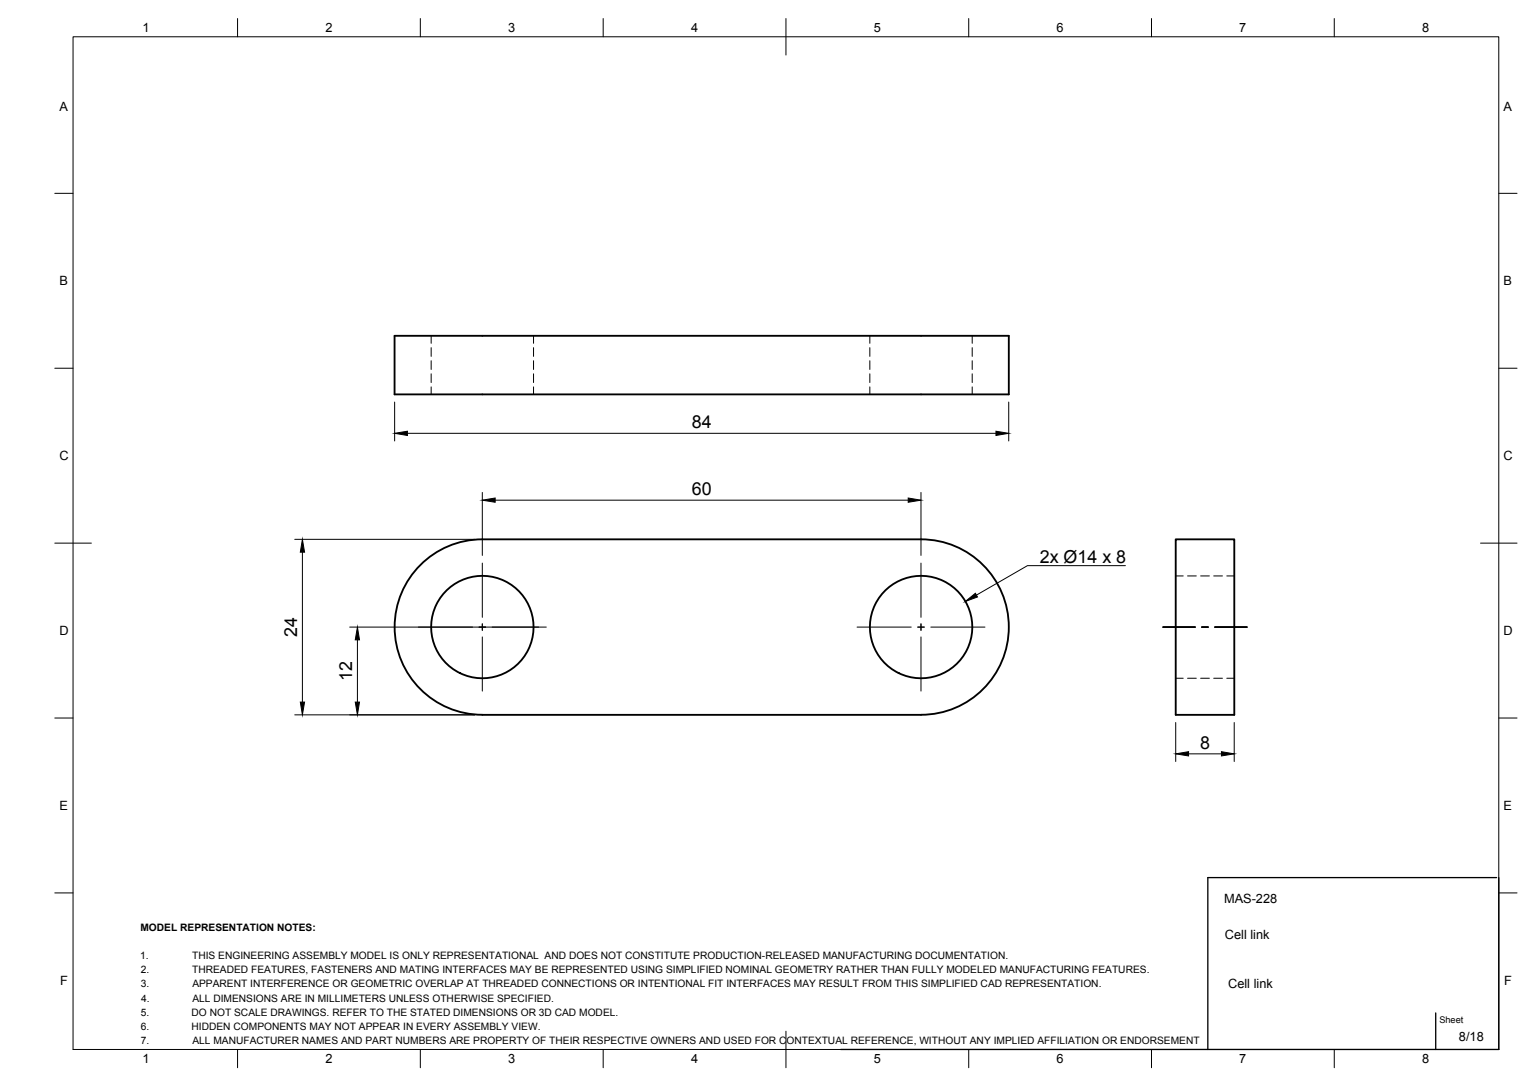
ISO-10303-21;
HEADER;
/* Generated by software containing ST-Developer
 * from STEP Tools, Inc. (www.steptools.com) 
 */

FILE_DESCRIPTION(
/* description */ ('Independent Peaucellier-Lipkin straight-line linkage. Radius arms 100
 mm, inversion-cell links 60 mm, crank radius and fixed-pivot spacing 
32 mm. Inversion constant 6400 mm squared, nominal output straight lin
e X=100 mm. Overhead bearing bridge clears the layered moving links. N
o accuracy or load rating assigned.'),
/* implementation_level */ '2;1');

FILE_NAME(
/* name */ 'Cell link.step',
/* time_stamp */ '2026-11-09T18:06:16-08:00',
/* author */ (''),
/* organization */ (''),
/* preprocessor_version */ 'ST-DEVELOPER v20.2',
/* originating_system */ 'Autodesk Translation Framework v15.17.0.0',
/* authorisation */ '');

FILE_SCHEMA (('AUTOMOTIVE_DESIGN { 1 0 10303 214 3 1 1 }'));
ENDSEC;

DATA;
#10=MECHANICAL_DESIGN_GEOMETRIC_PRESENTATION_REPRESENTATION('',(#288),#3581);
#254=SHAPE_REPRESENTATION_RELATIONSHIP('SRR','None',#3688,#271);
#271=ADVANCED_BREP_SHAPE_REPRESENTATION('',(#305),#3570);
#288=STYLED_ITEM('',(#3781),#305);
#305=MANIFOLD_SOLID_BREP('Body1',#1874);
#338=FACE_BOUND('',#606,.T.);
#339=FACE_BOUND('',#607,.T.);
#340=FACE_BOUND('',#609,.T.);
#341=FACE_BOUND('',#610,.T.);
#388=PLANE('',#2162);
#389=PLANE('',#2166);
#390=PLANE('',#2170);
#391=PLANE('',#2171);
#466=FACE_OUTER_BOUND('',#599,.T.);
#467=FACE_OUTER_BOUND('',#600,.T.);
#468=FACE_OUTER_BOUND('',#601,.T.);
#469=FACE_OUTER_BOUND('',#602,.T.);
#470=FACE_OUTER_BOUND('',#603,.T.);
#471=FACE_OUTER_BOUND('',#604,.T.);
#472=FACE_OUTER_BOUND('',#605,.T.);
#473=FACE_OUTER_BOUND('',#608,.T.);
#599=EDGE_LOOP('',(#1490,#1491,#1492,#1493));
#600=EDGE_LOOP('',(#1494,#1495,#1496,#1497));
#601=EDGE_LOOP('',(#1498,#1499,#1500,#1501));
#602=EDGE_LOOP('',(#1502,#1503,#1504,#1505));
#603=EDGE_LOOP('',(#1506,#1507,#1508,#1509));
#604=EDGE_LOOP('',(#1510,#1511,#1512,#1513));
#605=EDGE_LOOP('',(#1514,#1515,#1516,#1517));
#606=EDGE_LOOP('',(#1518));
#607=EDGE_LOOP('',(#1519));
#608=EDGE_LOOP('',(#1520,#1521,#1522,#1523));
#609=EDGE_LOOP('',(#1524));
#610=EDGE_LOOP('',(#1525));
#748=LINE('',#3227,#846);
#749=LINE('',#3233,#847);
#750=LINE('',#3238,#848);
#751=LINE('',#3240,#849);
#752=LINE('',#3242,#850);
#753=LINE('',#3243,#851);
#754=LINE('',#3249,#852);
#755=LINE('',#3252,#853);
#756=LINE('',#3254,#854);
#757=LINE('',#3255,#855);
#846=VECTOR('',#2582,7.);
#847=VECTOR('',#2589,7.);
#848=VECTOR('',#2594,10.);
#849=VECTOR('',#2595,10.);
#850=VECTOR('',#2596,10.);
#851=VECTOR('',#2597,10.);
#852=VECTOR('',#2604,10.);
#853=VECTOR('',#2607,10.);
#854=VECTOR('',#2608,10.);
#855=VECTOR('',#2609,10.);
#925=CIRCLE('',#2157,7.);
#926=CIRCLE('',#2158,7.);
#927=CIRCLE('',#2160,7.);
#928=CIRCLE('',#2161,7.);
#929=CIRCLE('',#2164,12.);
#930=CIRCLE('',#2165,12.);
#931=CIRCLE('',#2168,12.);
#932=CIRCLE('',#2169,12.);
#1047=VERTEX_POINT('',#3224);
#1048=VERTEX_POINT('',#3226);
#1049=VERTEX_POINT('',#3230);
#1050=VERTEX_POINT('',#3232);
#1051=VERTEX_POINT('',#3236);
#1052=VERTEX_POINT('',#3237);
#1053=VERTEX_POINT('',#3239);
#1054=VERTEX_POINT('',#3241);
#1055=VERTEX_POINT('',#3245);
#1056=VERTEX_POINT('',#3247);
#1057=VERTEX_POINT('',#3251);
#1058=VERTEX_POINT('',#3253);
#1207=EDGE_CURVE('',#1047,#1047,#925,.T.);
#1208=EDGE_CURVE('',#1047,#1048,#748,.T.);
#1209=EDGE_CURVE('',#1048,#1048,#926,.T.);
#1210=EDGE_CURVE('',#1049,#1049,#927,.T.);
#1211=EDGE_CURVE('',#1049,#1050,#749,.T.);
#1212=EDGE_CURVE('',#1050,#1050,#928,.T.);
#1213=EDGE_CURVE('',#1051,#1052,#750,.T.);
#1214=EDGE_CURVE('',#1052,#1053,#751,.T.);
#1215=EDGE_CURVE('',#1054,#1053,#752,.T.);
#1216=EDGE_CURVE('',#1051,#1054,#753,.T.);
#1217=EDGE_CURVE('',#1055,#1051,#929,.T.);
#1218=EDGE_CURVE('',#1056,#1054,#930,.T.);
#1219=EDGE_CURVE('',#1055,#1056,#754,.T.);
#1220=EDGE_CURVE('',#1057,#1055,#755,.T.);
#1221=EDGE_CURVE('',#1058,#1056,#756,.T.);
#1222=EDGE_CURVE('',#1057,#1058,#757,.T.);
#1223=EDGE_CURVE('',#1052,#1057,#931,.T.);
#1224=EDGE_CURVE('',#1053,#1058,#932,.T.);
#1490=ORIENTED_EDGE('',*,*,#1207,.F.);
#1491=ORIENTED_EDGE('',*,*,#1208,.T.);
#1492=ORIENTED_EDGE('',*,*,#1209,.F.);
#1493=ORIENTED_EDGE('',*,*,#1208,.F.);
#1494=ORIENTED_EDGE('',*,*,#1210,.F.);
#1495=ORIENTED_EDGE('',*,*,#1211,.T.);
#1496=ORIENTED_EDGE('',*,*,#1212,.F.);
#1497=ORIENTED_EDGE('',*,*,#1211,.F.);
#1498=ORIENTED_EDGE('',*,*,#1213,.T.);
#1499=ORIENTED_EDGE('',*,*,#1214,.T.);
#1500=ORIENTED_EDGE('',*,*,#1215,.F.);
#1501=ORIENTED_EDGE('',*,*,#1216,.F.);
#1502=ORIENTED_EDGE('',*,*,#1217,.T.);
#1503=ORIENTED_EDGE('',*,*,#1216,.T.);
#1504=ORIENTED_EDGE('',*,*,#1218,.F.);
#1505=ORIENTED_EDGE('',*,*,#1219,.F.);
#1506=ORIENTED_EDGE('',*,*,#1220,.T.);
#1507=ORIENTED_EDGE('',*,*,#1219,.T.);
#1508=ORIENTED_EDGE('',*,*,#1221,.F.);
#1509=ORIENTED_EDGE('',*,*,#1222,.F.);
#1510=ORIENTED_EDGE('',*,*,#1223,.T.);
#1511=ORIENTED_EDGE('',*,*,#1222,.T.);
#1512=ORIENTED_EDGE('',*,*,#1224,.F.);
#1513=ORIENTED_EDGE('',*,*,#1214,.F.);
#1514=ORIENTED_EDGE('',*,*,#1224,.T.);
#1515=ORIENTED_EDGE('',*,*,#1221,.T.);
#1516=ORIENTED_EDGE('',*,*,#1218,.T.);
#1517=ORIENTED_EDGE('',*,*,#1215,.T.);
#1518=ORIENTED_EDGE('',*,*,#1207,.T.);
#1519=ORIENTED_EDGE('',*,*,#1210,.T.);
#1520=ORIENTED_EDGE('',*,*,#1223,.F.);
#1521=ORIENTED_EDGE('',*,*,#1213,.F.);
#1522=ORIENTED_EDGE('',*,*,#1217,.F.);
#1523=ORIENTED_EDGE('',*,*,#1220,.F.);
#1524=ORIENTED_EDGE('',*,*,#1209,.T.);
#1525=ORIENTED_EDGE('',*,*,#1212,.T.);
#1725=CYLINDRICAL_SURFACE('',#2156,7.);
#1726=CYLINDRICAL_SURFACE('',#2159,7.);
#1727=CYLINDRICAL_SURFACE('',#2163,12.);
#1728=CYLINDRICAL_SURFACE('',#2167,12.);
#1798=ADVANCED_FACE('',(#466),#1725,.F.);
#1799=ADVANCED_FACE('',(#467),#1726,.F.);
#1800=ADVANCED_FACE('',(#468),#388,.T.);
#1801=ADVANCED_FACE('',(#469),#1727,.T.);
#1802=ADVANCED_FACE('',(#470),#389,.T.);
#1803=ADVANCED_FACE('',(#471),#1728,.T.);
#1804=ADVANCED_FACE('',(#472,#338,#339),#390,.T.);
#1805=ADVANCED_FACE('',(#473,#340,#341),#391,.F.);
#1874=CLOSED_SHELL('',(#1798,#1799,#1800,#1801,#1802,#1803,#1804,#1805));
#2155=AXIS2_PLACEMENT_3D('',#3222,#2576,#2577);
#2156=AXIS2_PLACEMENT_3D('',#3223,#2578,#2579);
#2157=AXIS2_PLACEMENT_3D('',#3225,#2580,#2581);
#2158=AXIS2_PLACEMENT_3D('',#3228,#2583,#2584);
#2159=AXIS2_PLACEMENT_3D('',#3229,#2585,#2586);
#2160=AXIS2_PLACEMENT_3D('',#3231,#2587,#2588);
#2161=AXIS2_PLACEMENT_3D('',#3234,#2590,#2591);
#2162=AXIS2_PLACEMENT_3D('',#3235,#2592,#2593);
#2163=AXIS2_PLACEMENT_3D('',#3244,#2598,#2599);
#2164=AXIS2_PLACEMENT_3D('',#3246,#2600,#2601);
#2165=AXIS2_PLACEMENT_3D('',#3248,#2602,#2603);
#2166=AXIS2_PLACEMENT_3D('',#3250,#2605,#2606);
#2167=AXIS2_PLACEMENT_3D('',#3256,#2610,#2611);
#2168=AXIS2_PLACEMENT_3D('',#3257,#2612,#2613);
#2169=AXIS2_PLACEMENT_3D('',#3258,#2614,#2615);
#2170=AXIS2_PLACEMENT_3D('',#3259,#2616,#2617);
#2171=AXIS2_PLACEMENT_3D('',#3260,#2618,#2619);
#2576=DIRECTION('axis',(0.,0.,1.));
#2577=DIRECTION('refdir',(1.,0.,0.));
#2578=DIRECTION('center_axis',(0.,0.,-1.));
#2579=DIRECTION('ref_axis',(1.,0.,0.));
#2580=DIRECTION('center_axis',(0.,0.,-1.));
#2581=DIRECTION('ref_axis',(1.,0.,0.));
#2582=DIRECTION('',(0.,0.,-1.));
#2583=DIRECTION('center_axis',(0.,0.,1.));
#2584=DIRECTION('ref_axis',(1.,0.,0.));
#2585=DIRECTION('center_axis',(0.,0.,-1.));
#2586=DIRECTION('ref_axis',(1.,0.,0.));
#2587=DIRECTION('center_axis',(0.,0.,-1.));
#2588=DIRECTION('ref_axis',(1.,0.,0.));
#2589=DIRECTION('',(0.,0.,-1.));
#2590=DIRECTION('center_axis',(0.,0.,1.));
#2591=DIRECTION('ref_axis',(1.,0.,0.));
#2592=DIRECTION('center_axis',(0.,1.,0.));
#2593=DIRECTION('ref_axis',(-1.,0.,0.));
#2594=DIRECTION('',(-1.,0.,0.));
#2595=DIRECTION('',(0.,0.,1.));
#2596=DIRECTION('',(-1.,0.,0.));
#2597=DIRECTION('',(0.,0.,1.));
#2598=DIRECTION('center_axis',(0.,0.,1.));
#2599=DIRECTION('ref_axis',(0.,-1.,0.));
#2600=DIRECTION('center_axis',(0.,0.,1.));
#2601=DIRECTION('ref_axis',(0.,-1.,0.));
#2602=DIRECTION('center_axis',(0.,0.,1.));
#2603=DIRECTION('ref_axis',(0.,-1.,0.));
#2604=DIRECTION('',(0.,0.,1.));
#2605=DIRECTION('center_axis',(0.,-1.,0.));
#2606=DIRECTION('ref_axis',(1.,0.,0.));
#2607=DIRECTION('',(1.,0.,0.));
#2608=DIRECTION('',(1.,0.,0.));
#2609=DIRECTION('',(0.,0.,1.));
#2610=DIRECTION('center_axis',(0.,0.,1.));
#2611=DIRECTION('ref_axis',(0.,1.,0.));
#2612=DIRECTION('center_axis',(0.,0.,1.));
#2613=DIRECTION('ref_axis',(0.,1.,0.));
#2614=DIRECTION('center_axis',(0.,0.,1.));
#2615=DIRECTION('ref_axis',(0.,1.,0.));
#2616=DIRECTION('center_axis',(0.,0.,1.));
#2617=DIRECTION('ref_axis',(1.,0.,0.));
#2618=DIRECTION('center_axis',(0.,0.,1.));
#2619=DIRECTION('ref_axis',(1.,0.,0.));
#3222=CARTESIAN_POINT('',(0.,0.,0.));
#3223=CARTESIAN_POINT('Origin',(0.,0.,4.));
#3224=CARTESIAN_POINT('',(-7.,8.57252759403147E-16,8.));
#3225=CARTESIAN_POINT('Origin',(0.,0.,8.));
#3226=CARTESIAN_POINT('',(-7.,8.57252759403147E-16,0.));
#3227=CARTESIAN_POINT('',(-7.,8.57252759403147E-16,4.));
#3228=CARTESIAN_POINT('Origin',(0.,0.,0.));
#3229=CARTESIAN_POINT('Origin',(60.,0.,4.));
#3230=CARTESIAN_POINT('',(53.,8.57252759403147E-16,8.));
#3231=CARTESIAN_POINT('Origin',(60.,0.,8.));
#3232=CARTESIAN_POINT('',(53.,8.57252759403147E-16,0.));
#3233=CARTESIAN_POINT('',(53.,8.57252759403147E-16,4.));
#3234=CARTESIAN_POINT('Origin',(60.,0.,0.));
#3235=CARTESIAN_POINT('Origin',(60.,12.,0.));
#3236=CARTESIAN_POINT('',(60.,12.,0.));
#3237=CARTESIAN_POINT('',(0.,12.,0.));
#3238=CARTESIAN_POINT('',(60.,12.,0.));
#3239=CARTESIAN_POINT('',(0.,12.,8.));
#3240=CARTESIAN_POINT('',(0.,12.,0.));
#3241=CARTESIAN_POINT('',(60.,12.,8.));
#3242=CARTESIAN_POINT('',(60.,12.,8.));
#3243=CARTESIAN_POINT('',(60.,12.,0.));
#3244=CARTESIAN_POINT('Origin',(60.,0.,0.));
#3245=CARTESIAN_POINT('',(60.,-12.,0.));
#3246=CARTESIAN_POINT('Origin',(60.,0.,0.));
#3247=CARTESIAN_POINT('',(60.,-12.,8.));
#3248=CARTESIAN_POINT('Origin',(60.,0.,8.));
#3249=CARTESIAN_POINT('',(60.,-12.,0.));
#3250=CARTESIAN_POINT('Origin',(0.,-12.,0.));
#3251=CARTESIAN_POINT('',(-1.46957615897682E-15,-12.,0.));
#3252=CARTESIAN_POINT('',(0.,-12.,0.));
#3253=CARTESIAN_POINT('',(-1.46957615897682E-15,-12.,8.));
#3254=CARTESIAN_POINT('',(0.,-12.,8.));
#3255=CARTESIAN_POINT('',(-1.46957615897682E-15,-12.,0.));
#3256=CARTESIAN_POINT('Origin',(0.,0.,0.));
#3257=CARTESIAN_POINT('Origin',(0.,0.,0.));
#3258=CARTESIAN_POINT('Origin',(0.,0.,8.));
#3259=CARTESIAN_POINT('Origin',(30.,0.,8.));
#3260=CARTESIAN_POINT('Origin',(30.,0.,0.));
#3551=UNCERTAINTY_MEASURE_WITH_UNIT(LENGTH_MEASURE(0.01),#3582,
'DISTANCE_ACCURACY_VALUE',
'Maximum model space distance between geometric entities at asserted c
onnectivities');
#3562=UNCERTAINTY_MEASURE_WITH_UNIT(LENGTH_MEASURE(0.01),#3582,
'DISTANCE_ACCURACY_VALUE',
'Maximum model space distance between geometric entities at asserted c
onnectivities');
#3570=(
GEOMETRIC_REPRESENTATION_CONTEXT(3)
GLOBAL_UNCERTAINTY_ASSIGNED_CONTEXT((#3551))
GLOBAL_UNIT_ASSIGNED_CONTEXT((#3582,#3584,#3585))
REPRESENTATION_CONTEXT('','3D')
);
#3581=(
GEOMETRIC_REPRESENTATION_CONTEXT(3)
GLOBAL_UNCERTAINTY_ASSIGNED_CONTEXT((#3562))
GLOBAL_UNIT_ASSIGNED_CONTEXT((#3582,#3584,#3585))
REPRESENTATION_CONTEXT('','3D')
);
#3582=(
LENGTH_UNIT()
NAMED_UNIT(*)
SI_UNIT(.MILLI.,.METRE.)
);
#3584=(
NAMED_UNIT(*)
PLANE_ANGLE_UNIT()
SI_UNIT($,.RADIAN.)
);
#3585=(
NAMED_UNIT(*)
SI_UNIT($,.STERADIAN.)
SOLID_ANGLE_UNIT()
);
#3593=SHAPE_DEFINITION_REPRESENTATION(#3611,#3688);
#3611=PRODUCT_DEFINITION_SHAPE('',$,#3707);
#3688=SHAPE_REPRESENTATION('',(#2155),#3570);
#3699=PRODUCT_DEFINITION_CONTEXT('part definition',#3755,'design');
#3707=PRODUCT_DEFINITION('Cell link','Cell link',#3725,#3699);
#3725=PRODUCT_DEFINITION_FORMATION('',$,#3764);
#3755=APPLICATION_CONTEXT(
'Core Data for Automotive Mechanical Design Process');
#3756=PRODUCT_CONTEXT('part definition',#3755,'mechanical');
#3764=PRODUCT('Cell link','Cell link',$,(#3756));
#3781=PRESENTATION_STYLE_ASSIGNMENT((#3794));
#3794=SURFACE_STYLE_USAGE(.BOTH.,#3807);
#3807=SURFACE_SIDE_STYLE('',(#3820));
#3820=SURFACE_STYLE_FILL_AREA(#3833);
#3833=FILL_AREA_STYLE('Cell link finish',(#3846));
#3846=FILL_AREA_STYLE_COLOUR('Cell link finish',#3859);
#3859=COLOUR_RGB('Cell link finish',0.317647058823529,0.686274509803922,
0.890196078431372);
ENDSEC;
END-ISO-10303-21;
